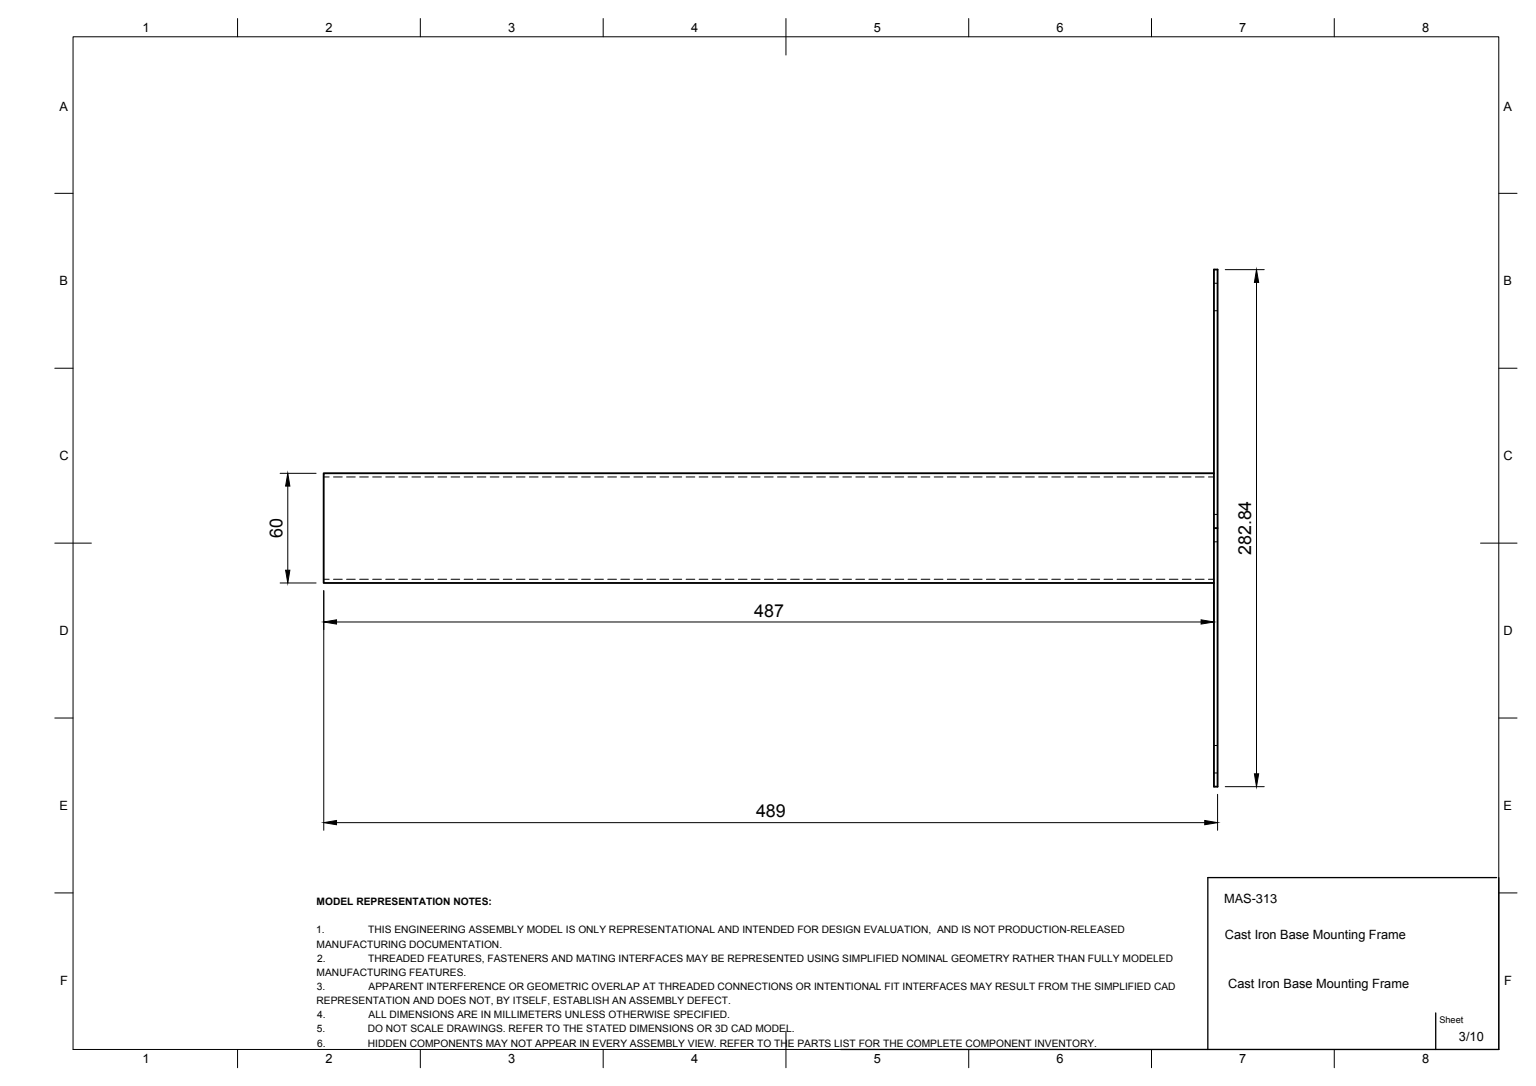
ISO-10303-21;
HEADER;
FILE_DESCRIPTION (('STEP AP214'),
    '1' );
FILE_NAME ('Cast Iron Base Mounting Frame.step',
    '2026-10-06T09:36:00',
    ( '' ),
    ( '' ),
    'SwSTEP 2.0',
    'SolidWorks 2025',
    '' );
FILE_SCHEMA (( 'AUTOMOTIVE_DESIGN' ));
ENDSEC;

DATA;
#2=ORIENTED_EDGE ( 'NONE', *, *, #7069, .T. ) ;
#13=CARTESIAN_POINT ( 'NONE',  ( -6.360897667028196044E-14, -494.9999999999998863, -141.4213562373094817 ) ) ;
#17=CYLINDRICAL_SURFACE ( 'NONE', #5203, 7.500000000000007105 ) ;
#40=DIRECTION ( 'NONE',  ( -6.195440985631454085E-17, 0.000000000000000000, 1.000000000000000000 ) ) ;
#61=CIRCLE ( 'NONE', #6581, 7.500000000000007105 ) ;
#73=LINE ( 'NONE', #6513, #3701 ) ;
#103=ORIENTED_EDGE ( 'NONE', *, *, #874, .T. ) ;
#112=DIRECTION ( 'NONE',  ( 1.000000000000000000, 0.000000000000000000, 0.000000000000000000 ) ) ;
#114=LINE ( 'NONE', #2966, #2548 ) ;
#160=AXIS2_PLACEMENT_3D ( 'NONE', #10271, #8167, #6559 ) ;
#171=CARTESIAN_POINT ( 'NONE',  ( -126.4213562373094959, -492.9999999999998863, 2.255140518769849223E-14 ) ) ;
#197=EDGE_LOOP ( 'NONE', ( #6499, #7897, #12076, #5197 ) ) ;
#203=ORIENTED_EDGE ( 'NONE', *, *, #874, .F. ) ;
#228=CARTESIAN_POINT ( 'NONE',  ( 0.000000000000000000, -494.9999999999998863, 0.000000000000000000 ) ) ;
#256=VECTOR ( 'NONE', #4482, 1000.000000000000000 ) ;
#258=LINE ( 'NONE', #2469, #6072 ) ;
#276=VECTOR ( 'NONE', #8146, 1000.000000000000000 ) ;
#358=ORIENTED_EDGE ( 'NONE', *, *, #9645, .T. ) ;
#376=CIRCLE ( 'NONE', #5908, 7.500000000000012434 ) ;
#381=DIRECTION ( 'NONE',  ( -0.000000000000000000, 1.000000000000000000, -0.000000000000000000 ) ) ;
#395=ORIENTED_EDGE ( 'NONE', *, *, #7971, .T. ) ;
#413=CARTESIAN_POINT ( 'NONE',  ( 1.387778780781445676E-14, -494.9999999999998863, 126.4213562373094959 ) ) ;
#429=CARTESIAN_POINT ( 'NONE',  ( 30.00000000000000000, -492.9999999999998863, -30.00000000000000000 ) ) ;
#436=FACE_OUTER_BOUND ( 'NONE', #2758, .T. ) ;
#507=CARTESIAN_POINT ( 'NONE',  ( -27.99999999999999645, -6.000000000000000000, 27.99999999999999645 ) ) ;
#510=PLANE ( 'NONE',  #8625 ) ;
#511=VECTOR ( 'NONE', #1443, 1000.000000000000000 ) ;
#532=VECTOR ( 'NONE', #8116, 1000.000000000000000 ) ;
#541=CARTESIAN_POINT ( 'NONE',  ( 4.808665244885994618E-14, -494.9999999999998863, 141.4213562373094817 ) ) ;
#558=SURFACE_STYLE_USAGE ( .BOTH. , #4395 ) ;
#565=FACE_OUTER_BOUND ( 'NONE', #10182, .T. ) ;
#577=CARTESIAN_POINT ( 'NONE',  ( 4.808665244885994618E-14, -492.9999999999998863, 141.4213562373094817 ) ) ;
#580=EDGE_CURVE ( 'NONE', #6384, #8630, #3180, .T. ) ;
#594=DIRECTION ( 'NONE',  ( -0.000000000000000000, 1.000000000000000000, -0.000000000000000000 ) ) ;
#623=FILL_AREA_STYLE ('',( #9083 ) ) ;
#628=ORIENTED_EDGE ( 'NONE', *, *, #11249, .F. ) ;
#657=LINE ( 'NONE', #9378, #2240 ) ;
#661=AXIS2_PLACEMENT_3D ( 'NONE', #11295, #2830, #6599 ) ;
#662=LINE ( 'NONE', #4437, #1336 ) ;
#665=DIRECTION ( 'NONE',  ( 0.7071067811865473507, 0.000000000000000000, -0.7071067811865477948 ) ) ;
#676=ORIENTED_EDGE ( 'NONE', *, *, #11233, .F. ) ;
#681=SURFACE_STYLE_FILL_AREA ( #9080 ) ;
#686=CARTESIAN_POINT ( 'NONE',  ( 1.387778780781445676E-14, -494.9999999999998863, 126.4213562373094959 ) ) ;
#706=CARTESIAN_POINT ( 'NONE',  ( 28.00000000000000000, -492.9999999999998863, -27.99999999999999645 ) ) ;
#730=EDGE_LOOP ( 'NONE', ( #10708, #628 ) ) ;
#752=( LENGTH_UNIT ( ) NAMED_UNIT ( * ) SI_UNIT ( .MILLI., .METRE. ) );
#755=DIRECTION ( 'NONE',  ( -0.000000000000000000, 1.000000000000000000, -0.000000000000000000 ) ) ;
#778=LINE ( 'NONE', #4551, #2867 ) ;
#781=DIRECTION ( 'NONE',  ( -0.000000000000000000, 1.000000000000000000, -0.000000000000000000 ) ) ;
#858=CARTESIAN_POINT ( 'NONE',  ( 141.4213562373095101, -494.9999999999998863, -1.508194112741312283E-14 ) ) ;
#874=EDGE_CURVE ( 'NONE', #6680, #11382, #2755, .T. ) ;
#882=VERTEX_POINT ( 'NONE', #9106 ) ;
#916=CARTESIAN_POINT ( 'NONE',  ( -27.99999999999999645, -492.9999999999998863, -27.99999999999999645 ) ) ;
#934=FACE_OUTER_BOUND ( 'NONE', #2126, .T. ) ;
#938=ORIENTED_EDGE ( 'NONE', *, *, #10249, .F. ) ;
#991=ORIENTED_EDGE ( 'NONE', *, *, #7995, .F. ) ;
#994=DIRECTION ( 'NONE',  ( 0.000000000000000000, -1.000000000000000000, 0.000000000000000000 ) ) ;
#1026=EDGE_CURVE ( 'NONE', #5299, #3186, #258, .T. ) ;
#1033=EDGE_LOOP ( 'NONE', ( #203, #3266, #1398, #1116 ) ) ;
#1034=AXIS2_PLACEMENT_3D ( 'NONE', #858, #4628, #3686 ) ;
#1048=ADVANCED_FACE ( 'NONE', ( #8799 ), #6941, .F. ) ;
#1055=CIRCLE ( 'NONE', #4008, 7.500000000000012434 ) ;
#1070=ORIENTED_EDGE ( 'NONE', *, *, #5111, .F. ) ;
#1081=ORIENTED_EDGE ( 'NONE', *, *, #7850, .T. ) ;
#1093=VECTOR ( 'NONE', #5863, 1000.000000000000000 ) ;
#1094=PRODUCT_CONTEXT ( 'NONE', #11592, 'mechanical' ) ;
#1095=VECTOR ( 'NONE', #2198, 1000.000000000000000 ) ;
#1116=ORIENTED_EDGE ( 'NONE', *, *, #10704, .F. ) ;
#1144=AXIS2_PLACEMENT_3D ( 'NONE', #1240, #7036, #2348 ) ;
#1159=STYLED_ITEM ( 'NONE', ( #3335 ), #8147 ) ;
#1160=CARTESIAN_POINT ( 'NONE',  ( -27.99999999999999645, -492.9999999999998863, -27.99999999999999645 ) ) ;
#1167=VERTEX_POINT ( 'NONE', #6427 ) ;
#1194=ORIENTED_EDGE ( 'NONE', *, *, #1790, .T. ) ;
#1207=CARTESIAN_POINT ( 'NONE',  ( 30.00000000000000000, -492.9999999999998863, 30.00000000000000000 ) ) ;
#1231=CIRCLE ( 'NONE', #8130, 7.500000000000007105 ) ;
#1236=FACE_BOUND ( 'NONE', #1923, .T. ) ;
#1238=CARTESIAN_POINT ( 'NONE',  ( -30.00000000000000000, -6.000000000000000000, 30.00000000000000000 ) ) ;
#1240=CARTESIAN_POINT ( 'NONE',  ( -126.4213562373094959, -494.9999999999998863, 2.255140518769849223E-14 ) ) ;
#1241=AXIS2_PLACEMENT_3D ( 'NONE', #6713, #7704, #3984 ) ;
#1245=LINE ( 'NONE', #6867, #3581 ) ;
#1255=CARTESIAN_POINT ( 'NONE',  ( 126.4213562373094959, -494.9999999999998863, 7.500000000000006217 ) ) ;
#1288=ORIENTED_EDGE ( 'NONE', *, *, #6220, .T. ) ;
#1334=DIRECTION ( 'NONE',  ( 0.000000000000000000, 0.000000000000000000, -1.000000000000000000 ) ) ;
#1336=VECTOR ( 'NONE', #3342, 1000.000000000000000 ) ;
#1342=VERTEX_POINT ( 'NONE', #7847 ) ;
#1349=( GEOMETRIC_REPRESENTATION_CONTEXT ( 3 ) GLOBAL_UNCERTAINTY_ASSIGNED_CONTEXT ( ( #11660 ) ) GLOBAL_UNIT_ASSIGNED_CONTEXT ( ( #752, #8169, #4338 ) ) REPRESENTATION_CONTEXT ( 'NONE', 'WORKASPACE' ) );
#1361=DIRECTION ( 'NONE',  ( -0.000000000000000000, 1.000000000000000000, -0.000000000000000000 ) ) ;
#1398=ORIENTED_EDGE ( 'NONE', *, *, #12116, .F. ) ;
#1443=DIRECTION ( 'NONE',  ( 1.000000000000000000, 0.000000000000000000, 0.000000000000000000 ) ) ;
#1450=VECTOR ( 'NONE', #6580, 1000.000000000000000 ) ;
#1463=VECTOR ( 'NONE', #10507, 1000.000000000000000 ) ;
#1470=LINE ( 'NONE', #4375, #276 ) ;
#1473=FACE_OUTER_BOUND ( 'NONE', #8723, .T. ) ;
#1477=LINE ( 'NONE', #11189, #6951 ) ;
#1480=EDGE_CURVE ( 'NONE', #6424, #6402, #662, .T. ) ;
#1481=DIRECTION ( 'NONE',  ( 0.000000000000000000, -1.000000000000000000, 0.000000000000000000 ) ) ;
#1495=EDGE_CURVE ( 'NONE', #2379, #1167, #5320, .T. ) ;
#1500=CARTESIAN_POINT ( 'NONE',  ( 1.387778780781445676E-14, -492.9999999999998863, 126.4213562373094959 ) ) ;
#1513=ORIENTED_EDGE ( 'NONE', *, *, #6743, .T. ) ;
#1514=CARTESIAN_POINT ( 'NONE',  ( 0.000000000000000000, -492.9999999999998863, 0.000000000000000000 ) ) ;
#1557=CARTESIAN_POINT ( 'NONE',  ( 4.808665244885994618E-14, -494.9999999999998863, 141.4213562373094817 ) ) ;
#1611=VERTEX_POINT ( 'NONE', #9641 ) ;
#1622=VERTEX_POINT ( 'NONE', #7855 ) ;
#1703=LINE ( 'NONE', #916, #11145 ) ;
#1735=VERTEX_POINT ( 'NONE', #12032 ) ;
#1737=ORIENTED_EDGE ( 'NONE', *, *, #7538, .T. ) ;
#1742=DIRECTION ( 'NONE',  ( -0.000000000000000000, 1.000000000000000000, -0.000000000000000000 ) ) ;
#1747=ORIENTED_EDGE ( 'NONE', *, *, #11277, .F. ) ;
#1790=EDGE_CURVE ( 'NONE', #7713, #882, #657, .T. ) ;
#1800=SURFACE_SIDE_STYLE ('',( #681 ) ) ;
#1817=ORIENTED_EDGE ( 'NONE', *, *, #9085, .F. ) ;
#1820=DIRECTION ( 'NONE',  ( 0.000000000000000000, 0.000000000000000000, -1.000000000000000000 ) ) ;
#1831=EDGE_LOOP ( 'NONE', ( #6682, #7432 ) ) ;
#1839=VECTOR ( 'NONE', #9227, 1000.000000000000000 ) ;
#1884=EDGE_CURVE ( 'NONE', #8131, #5617, #61, .T. ) ;
#1885=ORIENTED_EDGE ( 'NONE', *, *, #5319, .F. ) ;
#1917=DIRECTION ( 'NONE',  ( -0.000000000000000000, 0.000000000000000000, 1.000000000000000000 ) ) ;
#1921=CARTESIAN_POINT ( 'NONE',  ( 126.4213562373094959, -494.9999999999998863, -7.500000000000019540 ) ) ;
#1923=EDGE_LOOP ( 'NONE', ( #6325, #7312 ) ) ;
#1925=ORIENTED_EDGE ( 'NONE', *, *, #2302, .F. ) ;
#1928=DIRECTION ( 'NONE',  ( 0.000000000000000000, 0.000000000000000000, 1.000000000000000000 ) ) ;
#1941=DIRECTION ( 'NONE',  ( -0.7071067811865479058, 0.000000000000000000, -0.7071067811865472397 ) ) ;
#1963=DIRECTION ( 'NONE',  ( 0.000000000000000000, 0.000000000000000000, -1.000000000000000000 ) ) ;
#1970=CARTESIAN_POINT ( 'NONE',  ( 9.184850993605165694E-16, -494.9999999999998863, -133.9213562373095101 ) ) ;
#1982=DIRECTION ( 'NONE',  ( 0.000000000000000000, -0.000000000000000000, -1.000000000000000000 ) ) ;
#2015=VERTEX_POINT ( 'NONE', #9322 ) ;
#2037=FACE_BOUND ( 'NONE', #3887, .T. ) ;
#2060=DIRECTION ( 'NONE',  ( 0.7071067811865473507, 0.000000000000000000, -0.7071067811865477948 ) ) ;
#2061=VERTEX_POINT ( 'NONE', #1970 ) ;
#2067=VECTOR ( 'NONE', #10887, 1000.000000000000000 ) ;
#2083=ORIENTED_EDGE ( 'NONE', *, *, #9085, .T. ) ;
#2105=FACE_OUTER_BOUND ( 'NONE', #1033, .T. ) ;
#2120=CARTESIAN_POINT ( 'NONE',  ( -126.4213562373094959, -494.9999999999998863, 2.255140518769849223E-14 ) ) ;
#2122=VECTOR ( 'NONE', #2385, 999.9999999999998863 ) ;
#2126=EDGE_LOOP ( 'NONE', ( #1513, #11428, #1925, #8252 ) ) ;
#2138=ADVANCED_FACE ( 'NONE', ( #9503 ), #8580, .F. ) ;
#2141=VECTOR ( 'NONE', #2060, 999.9999999999998863 ) ;
#2153=AXIS2_PLACEMENT_3D ( 'NONE', #228, #994, #1982 ) ;
#2162=( GEOMETRIC_REPRESENTATION_CONTEXT ( 3 ) GLOBAL_UNCERTAINTY_ASSIGNED_CONTEXT ( ( #8812 ) ) GLOBAL_UNIT_ASSIGNED_CONTEXT ( ( #2722, #12126, #6304 ) ) REPRESENTATION_CONTEXT ( 'NONE', 'WORKASPACE' ) );
#2186=EDGE_LOOP ( 'NONE', ( #4571, #11548, #991, #8312 ) ) ;
#2198=DIRECTION ( 'NONE',  ( -0.000000000000000000, 1.000000000000000000, -0.000000000000000000 ) ) ;
#2240=VECTOR ( 'NONE', #11289, 1000.000000000000000 ) ;
#2247=CARTESIAN_POINT ( 'NONE',  ( -30.00000000000000000, -492.9999999999998863, -30.00000000000000000 ) ) ;
#2251=CARTESIAN_POINT ( 'NONE',  ( 126.4213562373094959, -492.9999999999998863, -6.938893903907228378E-15 ) ) ;
#2258=CIRCLE ( 'NONE', #5009, 7.500000000000012434 ) ;
#2267=EDGE_CURVE ( 'NONE', #3571, #7713, #9039, .T. ) ;
#2300=CARTESIAN_POINT ( 'NONE',  ( 28.00000000000000000, -492.9999999999998863, -27.99999999999999645 ) ) ;
#2302=EDGE_CURVE ( 'NONE', #6384, #5463, #8505, .T. ) ;
#2345=AXIS2_PLACEMENT_3D ( 'NONE', #1500, #10714, #5261 ) ;
#2348=DIRECTION ( 'NONE',  ( 0.000000000000000000, 0.000000000000000000, 1.000000000000000000 ) ) ;
#2379=VERTEX_POINT ( 'NONE', #13 ) ;
#2385=DIRECTION ( 'NONE',  ( 0.7071067811865479058, 0.000000000000000000, 0.7071067811865472397 ) ) ;
#2402=DIRECTION ( 'NONE',  ( -0.7071067811865473507, 0.000000000000000000, 0.7071067811865477948 ) ) ;
#2449=AXIS2_PLACEMENT_3D ( 'NONE', #4231, #4414, #1334 ) ;
#2469=CARTESIAN_POINT ( 'NONE',  ( 1.387778780781445676E-14, -494.9999999999998863, 133.9213562373095101 ) ) ;
#2548=VECTOR ( 'NONE', #6729, 1000.000000000000000 ) ;
#2554=CARTESIAN_POINT ( 'NONE',  ( 1.479627290717497352E-14, -494.9999999999998863, 118.9213562373094817 ) ) ;
#2562=CARTESIAN_POINT ( 'NONE',  ( 1.387778780781445676E-14, -494.9999999999998863, 126.4213562373094959 ) ) ;
#2586=DIRECTION ( 'NONE',  ( -0.000000000000000000, 1.000000000000000000, -0.000000000000000000 ) ) ;
#2591=CYLINDRICAL_SURFACE ( 'NONE', #8082, 7.500000000000007105 ) ;
#2627=CARTESIAN_POINT ( 'NONE',  ( -30.00000000000000000, -492.9999999999998863, 30.00000000000000000 ) ) ;
#2658=AXIS2_PLACEMENT_3D ( 'NONE', #4296, #3402, #8912 ) ;
#2662=FACE_BOUND ( 'NONE', #3396, .T. ) ;
#2674=CARTESIAN_POINT ( 'NONE',  ( -27.99999999999999645, -492.9999999999998863, -27.99999999999999645 ) ) ;
#2722=( LENGTH_UNIT ( ) NAMED_UNIT ( * ) SI_UNIT ( .MILLI., .METRE. ) );
#2745=VECTOR ( 'NONE', #11263, 1000.000000000000000 ) ;
#2755=LINE ( 'NONE', #5335, #9899 ) ;
#2758=EDGE_LOOP ( 'NONE', ( #6588, #8120, #3553, #10029 ) ) ;
#2796=EDGE_LOOP ( 'NONE', ( #4764, #9890, #7885, #7728 ) ) ;
#2830=DIRECTION ( 'NONE',  ( -0.000000000000000000, 1.000000000000000000, -0.000000000000000000 ) ) ;
#2860=FACE_OUTER_BOUND ( 'NONE', #11455, .T. ) ;
#2867=VECTOR ( 'NONE', #10231, 1000.000000000000000 ) ;
#2878=DIRECTION ( 'NONE',  ( -0.000000000000000000, 1.000000000000000000, -0.000000000000000000 ) ) ;
#2885=LINE ( 'NONE', #9490, #11176 ) ;
#2886=DIRECTION ( 'NONE',  ( 0.000000000000000000, -1.000000000000000000, 0.000000000000000000 ) ) ;
#2892=( GEOMETRIC_REPRESENTATION_CONTEXT ( 3 ) GLOBAL_UNCERTAINTY_ASSIGNED_CONTEXT ( ( #9795 ) ) GLOBAL_UNIT_ASSIGNED_CONTEXT ( ( #4176, #6096, #3300 ) ) REPRESENTATION_CONTEXT ( 'NONE', 'WORKASPACE' ) );
#2910=PLANE ( 'NONE',  #10244 ) ;
#2912=PLANE ( 'NONE',  #3232 ) ;
#2919=EDGE_LOOP ( 'NONE', ( #12184, #7238, #7706, #2 ) ) ;
#2966=CARTESIAN_POINT ( 'NONE',  ( 141.4213562373095101, -494.9999999999998863, -1.508194112741312283E-14 ) ) ;
#2973=CARTESIAN_POINT ( 'NONE',  ( 1.387778780781445676E-14, -494.9999999999998863, 126.4213562373094959 ) ) ;
#3032=ORIENTED_EDGE ( 'NONE', *, *, #6284, .F. ) ;
#3043=ORIENTED_EDGE ( 'NONE', *, *, #9421, .F. ) ;
#3060=VECTOR ( 'NONE', #8488, 1000.000000000000000 ) ;
#3086=VECTOR ( 'NONE', #6084, 1000.000000000000000 ) ;
#3131=EDGE_LOOP ( 'NONE', ( #3257, #6840, #1194, #11050 ) ) ;
#3139=COLOUR_RGB ( '', 0.66274510, 0.83137255, 0.94901961) ;
#3143=PRODUCT_DEFINITION ( 'UNKNOWN', '', #3878, #11351 ) ;
#3180=LINE ( 'NONE', #5271, #7532 ) ;
#3186=VERTEX_POINT ( 'NONE', #5560 ) ;
#3200=DIRECTION ( 'NONE',  ( 0.000000000000000000, 0.000000000000000000, 1.000000000000000000 ) ) ;
#3232=AXIS2_PLACEMENT_3D ( 'NONE', #11313, #10567, #3892 ) ;
#3257=ORIENTED_EDGE ( 'NONE', *, *, #4672, .F. ) ;
#3266=ORIENTED_EDGE ( 'NONE', *, *, #10375, .F. ) ;
#3273=CARTESIAN_POINT ( 'NONE',  ( 0.000000000000000000, -492.9999999999998863, -126.4213562373094959 ) ) ;
#3279=ORIENTED_EDGE ( 'NONE', *, *, #6743, .F. ) ;
#3289=ADVANCED_FACE ( 'NONE', ( #934 ), #4706, .F. ) ;
#3294=CARTESIAN_POINT ( 'NONE',  ( -27.99999999999999645, -492.9999999999998863, -27.99999999999999645 ) ) ;
#3298=EDGE_LOOP ( 'NONE', ( #1885, #8268, #8263, #10866 ) ) ;
#3300=( NAMED_UNIT ( * ) SI_UNIT ( $, .STERADIAN. ) SOLID_ANGLE_UNIT ( ) );
#3303=DIRECTION ( 'NONE',  ( 0.000000000000000000, -1.000000000000000000, 0.000000000000000000 ) ) ;
#3317=CARTESIAN_POINT ( 'NONE',  ( 30.00000000000000000, -6.000000000000000000, 30.00000000000000000 ) ) ;
#3324=STYLED_ITEM ( 'NONE', ( #9337 ), #3758 ) ;
#3335=PRESENTATION_STYLE_ASSIGNMENT (( #558 ) ) ;
#3342=DIRECTION ( 'NONE',  ( -0.000000000000000000, 1.000000000000000000, -0.000000000000000000 ) ) ;
#3343=CARTESIAN_POINT ( 'NONE',  ( 28.00000000000000000, -492.9999999999998863, -27.99999999999999645 ) ) ;
#3367=AXIS2_PLACEMENT_3D ( 'NONE', #11658, #6029, #9911 ) ;
#3373=DIRECTION ( 'NONE',  ( 0.7071067811865477948, 0.000000000000000000, 0.7071067811865473507 ) ) ;
#3376=AXIS2_PLACEMENT_3D ( 'NONE', #4147, #5182, #6056 ) ;
#3389=ORIENTED_EDGE ( 'NONE', *, *, #5441, .F. ) ;
#3393=ADVANCED_FACE ( 'NONE', ( #2037, #4871, #9456, #3826, #4934 ), #9578, .T. ) ;
#3394=DIRECTION ( 'NONE',  ( 0.000000000000000000, 0.000000000000000000, 1.000000000000000000 ) ) ;
#3396=EDGE_LOOP ( 'NONE', ( #10120, #11963, #11935, #1737 ) ) ;
#3402=DIRECTION ( 'NONE',  ( 0.000000000000000000, -1.000000000000000000, 0.000000000000000000 ) ) ;
#3414=CARTESIAN_POINT ( 'NONE',  ( 1.387778780781445676E-14, -492.9999999999998863, 126.4213562373094959 ) ) ;
#3437=ADVANCED_FACE ( 'NONE', ( #2105, #11370, #6857, #8771, #1236 ), #2910, .F. ) ;
#3439=VECTOR ( 'NONE', #4347, 1000.000000000000000 ) ;
#3445=ORIENTED_EDGE ( 'NONE', *, *, #2302, .T. ) ;
#3458=ORIENTED_EDGE ( 'NONE', *, *, #1480, .T. ) ;
#3466=CIRCLE ( 'NONE', #6450, 7.500000000000012434 ) ;
#3470=CARTESIAN_POINT ( 'NONE',  ( 30.00000000000000000, -6.000000000000000000, -30.00000000000000000 ) ) ;
#3553=ORIENTED_EDGE ( 'NONE', *, *, #2267, .T. ) ;
#3571=VERTEX_POINT ( 'NONE', #8935 ) ;
#3581=VECTOR ( 'NONE', #11319, 1000.000000000000000 ) ;
#3588=LINE ( 'NONE', #2674, #1839 ) ;
#3601=SHAPE_REPRESENTATION ( 'Cast Iron Base Mounting Frame', ( #11957 ), #2892 ) ;
#3619=CARTESIAN_POINT ( 'NONE',  ( 4.808665244885994618E-14, -494.9999999999998863, 141.4213562373094817 ) ) ;
#3686=DIRECTION ( 'NONE',  ( -0.7071067811865473507, 0.000000000000000000, 0.7071067811865477948 ) ) ;
#3700=ORIENTED_EDGE ( 'NONE', *, *, #10907, .F. ) ;
#3701=VECTOR ( 'NONE', #3851, 999.9999999999998863 ) ;
#3754=ADVANCED_FACE ( 'NONE', ( #4334 ), #2591, .F. ) ;
#3758=MANIFOLD_SOLID_BREP ( 'Boss-Extrude7', #9857 ) ;
#3777=ORIENTED_EDGE ( 'NONE', *, *, #7850, .F. ) ;
#3815=ORIENTED_EDGE ( 'NONE', *, *, #7386, .T. ) ;
#3826=FACE_BOUND ( 'NONE', #7708, .T. ) ;
#3830=ADVANCED_BREP_SHAPE_REPRESENTATION ( '', ( #3758, #8147, #11957 ), #2892 ) ;
#3838=EDGE_LOOP ( 'NONE', ( #9982, #11366, #11265, #4376 ) ) ;
#3851=DIRECTION ( 'NONE',  ( 0.7071067811865479058, 0.000000000000000000, 0.7071067811865472397 ) ) ;
#3869=LINE ( 'NONE', #7761, #8276 ) ;
#3878=PRODUCT_DEFINITION_FORMATION_WITH_SPECIFIED_SOURCE ( 'ANY', '', #8619, .NOT_KNOWN. ) ;
#3879=ORIENTED_EDGE ( 'NONE', *, *, #1026, .F. ) ;
#3887=EDGE_LOOP ( 'NONE', ( #9683, #1817 ) ) ;
#3892=DIRECTION ( 'NONE',  ( -1.000000000000000000, 0.000000000000000000, -6.195440985631454085E-17 ) ) ;
#3893=ORIENTED_EDGE ( 'NONE', *, *, #5543, .T. ) ;
#3917=ORIENTED_EDGE ( 'NONE', *, *, #9408, .T. ) ;
#3918=EDGE_LOOP ( 'NONE', ( #5642, #3917 ) ) ;
#3922=ORIENTED_EDGE ( 'NONE', *, *, #6903, .F. ) ;
#3959=EDGE_CURVE ( 'NONE', #10867, #6680, #114, .T. ) ;
#3978=EDGE_CURVE ( 'NONE', #6402, #8803, #376, .T. ) ;
#3984=DIRECTION ( 'NONE',  ( 0.000000000000000000, 0.000000000000000000, -1.000000000000000000 ) ) ;
#4008=AXIS2_PLACEMENT_3D ( 'NONE', #2251, #10833, #6020 ) ;
#4080=VECTOR ( 'NONE', #381, 1000.000000000000000 ) ;
#4123=EDGE_CURVE ( 'NONE', #3186, #1611, #8088, .T. ) ;
#4124=ORIENTED_EDGE ( 'NONE', *, *, #6843, .F. ) ;
#4147=CARTESIAN_POINT ( 'NONE',  ( -126.4213562373094959, -494.9999999999998863, 2.255140518769849223E-14 ) ) ;
#4176=( LENGTH_UNIT ( ) NAMED_UNIT ( * ) SI_UNIT ( .MILLI., .METRE. ) );
#4221=CARTESIAN_POINT ( 'NONE',  ( 141.4213562373095101, -494.9999999999998863, -1.508194112741312283E-14 ) ) ;
#4231=CARTESIAN_POINT ( 'NONE',  ( 0.000000000000000000, -494.9999999999998863, -126.4213562373094959 ) ) ;
#4233=LINE ( 'NONE', #3294, #511 ) ;
#4239=AXIS2_PLACEMENT_3D ( 'NONE', #11561, #3303, #5162 ) ;
#4296=CARTESIAN_POINT ( 'NONE',  ( -126.4213562373094959, -492.9999999999998863, 2.255140518769849223E-14 ) ) ;
#4305=FACE_BOUND ( 'NONE', #197, .T. ) ;
#4321=AXIS2_PLACEMENT_3D ( 'NONE', #686, #6436, #8367 ) ;
#4334=FACE_OUTER_BOUND ( 'NONE', #8748, .T. ) ;
#4338=( NAMED_UNIT ( * ) SI_UNIT ( $, .STERADIAN. ) SOLID_ANGLE_UNIT ( ) );
#4345=CYLINDRICAL_SURFACE ( 'NONE', #8030, 7.500000000000012434 ) ;
#4347=DIRECTION ( 'NONE',  ( -0.000000000000000000, -0.000000000000000000, -1.000000000000000000 ) ) ;
#4359=CARTESIAN_POINT ( 'NONE',  ( 28.00000000000000000, -6.000000000000000000, -27.99999999999999645 ) ) ;
#4365=ORIENTED_EDGE ( 'NONE', *, *, #10907, .T. ) ;
#4375=CARTESIAN_POINT ( 'NONE',  ( -27.99999999999999645, -6.000000000000000000, -27.99999999999999645 ) ) ;
#4376=ORIENTED_EDGE ( 'NONE', *, *, #10779, .T. ) ;
#4395=SURFACE_SIDE_STYLE ('',( #10877 ) ) ;
#4401=EDGE_CURVE ( 'NONE', #4868, #10168, #11965, .T. ) ;
#4414=DIRECTION ( 'NONE',  ( 0.000000000000000000, -1.000000000000000000, 0.000000000000000000 ) ) ;
#4437=CARTESIAN_POINT ( 'NONE',  ( -126.4213562373094959, -494.9999999999998863, -7.499999999999990230 ) ) ;
#4442=LINE ( 'NONE', #11916, #5050 ) ;
#4459=ORIENTED_EDGE ( 'NONE', *, *, #1495, .F. ) ;
#4482=DIRECTION ( 'NONE',  ( -6.195440985631455317E-17, 0.000000000000000000, 1.000000000000000000 ) ) ;
#4503=ORIENTED_EDGE ( 'NONE', *, *, #8108, .F. ) ;
#4505=FACE_OUTER_BOUND ( 'NONE', #3838, .T. ) ;
#4508=FACE_OUTER_BOUND ( 'NONE', #5762, .T. ) ;
#4512=EDGE_CURVE ( 'NONE', #882, #10332, #3869, .T. ) ;
#4528=ORIENTED_EDGE ( 'NONE', *, *, #6284, .T. ) ;
#4539=LINE ( 'NONE', #1557, #532 ) ;
#4551=CARTESIAN_POINT ( 'NONE',  ( 30.00000000000000000, -492.9999999999998863, -30.00000000000000000 ) ) ;
#4571=ORIENTED_EDGE ( 'NONE', *, *, #10375, .T. ) ;
#4576=CARTESIAN_POINT ( 'NONE',  ( -141.4213562373095101, -494.9999999999998863, 3.644282033693712520E-14 ) ) ;
#4581=VERTEX_POINT ( 'NONE', #1160 ) ;
#4628=DIRECTION ( 'NONE',  ( -0.7071067811865477948, 0.000000000000000000, -0.7071067811865473507 ) ) ;
#4642=AXIS2_PLACEMENT_3D ( 'NONE', #3414, #6154, #8075 ) ;
#4645=EDGE_CURVE ( 'NONE', #1342, #2015, #6742, .T. ) ;
#4653=VECTOR ( 'NONE', #5823, 1000.000000000000000 ) ;
#4662=ORIENTED_EDGE ( 'NONE', *, *, #580, .F. ) ;
#4672=EDGE_CURVE ( 'NONE', #9067, #10332, #7843, .T. ) ;
#4706=PLANE ( 'NONE',  #12225 ) ;
#4725=LINE ( 'NONE', #5817, #5195 ) ;
#4728=LINE ( 'NONE', #11220, #11006 ) ;
#4739=ORIENTED_EDGE ( 'NONE', *, *, #4401, .F. ) ;
#4764=ORIENTED_EDGE ( 'NONE', *, *, #5752, .T. ) ;
#4785=CIRCLE ( 'NONE', #3376, 7.500000000000012434 ) ;
#4866=ADVANCED_FACE ( 'NONE', ( #12170 ), #11241, .F. ) ;
#4868=VERTEX_POINT ( 'NONE', #8406 ) ;
#4871=FACE_BOUND ( 'NONE', #730, .T. ) ;
#4889=MECHANICAL_DESIGN_GEOMETRIC_PRESENTATION_REPRESENTATION('',(#1159),#1349);
#4934=FACE_BOUND ( 'NONE', #8354, .T. ) ;
#4952=ADVANCED_FACE ( 'NONE', ( #5180 ), #7918, .F. ) ;
#4970=EDGE_LOOP ( 'NONE', ( #7452, #395, #1081, #10447 ) ) ;
#4994=DIRECTION ( 'NONE',  ( -1.000000000000000000, -0.000000000000000000, -0.000000000000000000 ) ) ;
#5009=AXIS2_PLACEMENT_3D ( 'NONE', #2120, #5879, #9658 ) ;
#5045=CARTESIAN_POINT ( 'NONE',  ( -27.99999999999999645, -6.000000000000000000, 27.99999999999999645 ) ) ;
#5050=VECTOR ( 'NONE', #10988, 1000.000000000000000 ) ;
#5059=LINE ( 'NONE', #7104, #9328 ) ;
#5062=ORIENTED_EDGE ( 'NONE', *, *, #1884, .T. ) ;
#5072=LINE ( 'NONE', #5881, #6076 ) ;
#5077=LINE ( 'NONE', #429, #4080 ) ;
#5111=EDGE_CURVE ( 'NONE', #10867, #11480, #1477, .T. ) ;
#5139=ORIENTED_EDGE ( 'NONE', *, *, #11277, .T. ) ;
#5143=ORIENTED_EDGE ( 'NONE', *, *, #9340, .F. ) ;
#5156=ADVANCED_FACE ( 'NONE', ( #4508 ), #6237, .F. ) ;
#5162=DIRECTION ( 'NONE',  ( 0.000000000000000000, 0.000000000000000000, -1.000000000000000000 ) ) ;
#5180=FACE_OUTER_BOUND ( 'NONE', #6618, .T. ) ;
#5182=DIRECTION ( 'NONE',  ( 0.000000000000000000, -1.000000000000000000, 0.000000000000000000 ) ) ;
#5193=VERTEX_POINT ( 'NONE', #4576 ) ;
#5195=VECTOR ( 'NONE', #7622, 1000.000000000000000 ) ;
#5197=ORIENTED_EDGE ( 'NONE', *, *, #9793, .F. ) ;
#5203=AXIS2_PLACEMENT_3D ( 'NONE', #5766, #2878, #5891 ) ;
#5261=DIRECTION ( 'NONE',  ( 0.000000000000000000, 0.000000000000000000, -1.000000000000000000 ) ) ;
#5264=FACE_OUTER_BOUND ( 'NONE', #8950, .T. ) ;
#5271=CARTESIAN_POINT ( 'NONE',  ( -30.00000000000000000, -492.9999999999998863, -30.00000000000000000 ) ) ;
#5276=DIRECTION ( 'NONE',  ( 0.000000000000000000, 1.000000000000000000, 0.000000000000000000 ) ) ;
#5289=PLANE ( 'NONE',  #9372 ) ;
#5299=VERTEX_POINT ( 'NONE', #9587 ) ;
#5307=ADVANCED_FACE ( 'NONE', ( #2860 ), #8543, .F. ) ;
#5319=EDGE_CURVE ( 'NONE', #6347, #10683, #1245, .T. ) ;
#5320=LINE ( 'NONE', #9965, #5588 ) ;
#5328=PLANE ( 'NONE',  #5675 ) ;
#5335=CARTESIAN_POINT ( 'NONE',  ( 141.4213562373095101, -492.9999999999998863, -1.508194112741312283E-14 ) ) ;
#5441=EDGE_CURVE ( 'NONE', #11262, #9215, #5059, .T. ) ;
#5463=VERTEX_POINT ( 'NONE', #8040 ) ;
#5474=AXIS2_PLACEMENT_3D ( 'NONE', #2247, #11990, #9782 ) ;
#5488=ADVANCED_FACE ( 'NONE', ( #7041 ), #8889, .F. ) ;
#5509=ORIENTED_EDGE ( 'NONE', *, *, #8908, .F. ) ;
#5525=CARTESIAN_POINT ( 'NONE',  ( -30.00000000000000000, -492.9999999999998863, -30.00000000000000000 ) ) ;
#5543=EDGE_CURVE ( 'NONE', #6424, #1735, #4785, .T. ) ;
#5555=EDGE_CURVE ( 'NONE', #5299, #7650, #1231, .T. ) ;
#5560=CARTESIAN_POINT ( 'NONE',  ( 1.387778780781445676E-14, -492.9999999999998863, 133.9213562373095101 ) ) ;
#5562=SURFACE_STYLE_USAGE ( .BOTH. , #1800 ) ;
#5588=VECTOR ( 'NONE', #7185, 1000.000000000000000 ) ;
#5608=EDGE_LOOP ( 'NONE', ( #103, #11015, #1070, #9434 ) ) ;
#5617=VERTEX_POINT ( 'NONE', #12101 ) ;
#5642=ORIENTED_EDGE ( 'NONE', *, *, #5852, .T. ) ;
#5675=AXIS2_PLACEMENT_3D ( 'NONE', #7255, #1820, #7685 ) ;
#5718=DIRECTION ( 'NONE',  ( 0.000000000000000000, 0.000000000000000000, -1.000000000000000000 ) ) ;
#5739=DIRECTION ( 'NONE',  ( 0.000000000000000000, -0.000000000000000000, -1.000000000000000000 ) ) ;
#5743=CARTESIAN_POINT ( 'NONE',  ( 141.4213562373095101, -492.9999999999998863, -1.508194112741312283E-14 ) ) ;
#5752=EDGE_CURVE ( 'NONE', #11517, #2061, #8361, .T. ) ;
#5761=AXIS2_PLACEMENT_3D ( 'NONE', #11982, #3373, #10929 ) ;
#5762=EDGE_LOOP ( 'NONE', ( #10342, #4459, #3777, #1288 ) ) ;
#5766=CARTESIAN_POINT ( 'NONE',  ( 0.000000000000000000, -494.9999999999998863, -126.4213562373094959 ) ) ;
#5770=CARTESIAN_POINT ( 'NONE',  ( -126.4213562373094959, -492.9999999999998863, 7.500000000000035527 ) ) ;
#5787=CARTESIAN_POINT ( 'NONE',  ( -30.00000000000000000, -6.000000000000000000, -30.00000000000000000 ) ) ;
#5817=CARTESIAN_POINT ( 'NONE',  ( -141.4213562373095101, -494.9999999999998863, 3.644282033693712520E-14 ) ) ;
#5822=VECTOR ( 'NONE', #4994, 1000.000000000000000 ) ;
#5823=DIRECTION ( 'NONE',  ( -0.000000000000000000, 1.000000000000000000, -0.000000000000000000 ) ) ;
#5825=ORIENTED_EDGE ( 'NONE', *, *, #5543, .F. ) ;
#5831=LINE ( 'NONE', #10654, #11552 ) ;
#5840=DIRECTION ( 'NONE',  ( -0.000000000000000000, 1.000000000000000000, -0.000000000000000000 ) ) ;
#5852=EDGE_CURVE ( 'NONE', #7207, #1622, #1055, .T. ) ;
#5863=DIRECTION ( 'NONE',  ( 1.000000000000000000, 0.000000000000000000, 0.000000000000000000 ) ) ;
#5879=DIRECTION ( 'NONE',  ( 0.000000000000000000, -1.000000000000000000, 0.000000000000000000 ) ) ;
#5881=CARTESIAN_POINT ( 'NONE',  ( 9.184850993605161750E-16, -494.9999999999998863, -133.9213562373095101 ) ) ;
#5891=DIRECTION ( 'NONE',  ( 0.000000000000000000, 0.000000000000000000, 1.000000000000000000 ) ) ;
#5895=DIRECTION ( 'NONE',  ( -6.195440985631455317E-17, 0.000000000000000000, 1.000000000000000000 ) ) ;
#5908=AXIS2_PLACEMENT_3D ( 'NONE', #171, #7720, #11495 ) ;
#5974=ORIENTED_EDGE ( 'NONE', *, *, #8854, .F. ) ;
#6004=AXIS2_PLACEMENT_3D ( 'NONE', #9338, #12192, #9143 ) ;
#6009=PLANE ( 'NONE',  #10594 ) ;
#6017=LINE ( 'NONE', #3343, #2067 ) ;
#6020=DIRECTION ( 'NONE',  ( 0.000000000000000000, 0.000000000000000000, -1.000000000000000000 ) ) ;
#6029=DIRECTION ( 'NONE',  ( 0.000000000000000000, -1.000000000000000000, 0.000000000000000000 ) ) ;
#6031=EDGE_CURVE ( 'NONE', #882, #4581, #3588, .T. ) ;
#6056=DIRECTION ( 'NONE',  ( 0.000000000000000000, 0.000000000000000000, -1.000000000000000000 ) ) ;
#6072=VECTOR ( 'NONE', #2586, 1000.000000000000000 ) ;
#6076=VECTOR ( 'NONE', #8848, 1000.000000000000000 ) ;
#6084=DIRECTION ( 'NONE',  ( -0.000000000000000000, 1.000000000000000000, -0.000000000000000000 ) ) ;
#6096=( NAMED_UNIT ( * ) PLANE_ANGLE_UNIT ( ) SI_UNIT ( $, .RADIAN. ) );
#6139=ORIENTED_EDGE ( 'NONE', *, *, #5441, .T. ) ;
#6154=DIRECTION ( 'NONE',  ( 0.000000000000000000, -1.000000000000000000, 0.000000000000000000 ) ) ;
#6194=ORIENTED_EDGE ( 'NONE', *, *, #4401, .T. ) ;
#6204=ORIENTED_EDGE ( 'NONE', *, *, #9340, .T. ) ;
#6220=EDGE_CURVE ( 'NONE', #5193, #7316, #4725, .T. ) ;
#6237=PLANE ( 'NONE',  #5761 ) ;
#6248=DIRECTION ( 'NONE',  ( 0.000000000000000000, 0.000000000000000000, 1.000000000000000000 ) ) ;
#6271=CARTESIAN_POINT ( 'NONE',  ( 4.808665244885994618E-14, -492.9999999999998863, 141.4213562373094817 ) ) ;
#6284=EDGE_CURVE ( 'NONE', #1735, #6424, #2258, .T. ) ;
#6304=( NAMED_UNIT ( * ) SI_UNIT ( $, .STERADIAN. ) SOLID_ANGLE_UNIT ( ) );
#6325=ORIENTED_EDGE ( 'NONE', *, *, #11233, .T. ) ;
#6347=VERTEX_POINT ( 'NONE', #11760 ) ;
#6364=FACE_OUTER_BOUND ( 'NONE', #3131, .T. ) ;
#6368=CARTESIAN_POINT ( 'NONE',  ( 0.000000000000000000, -492.9999999999998863, -118.9213562373094817 ) ) ;
#6384=VERTEX_POINT ( 'NONE', #10943 ) ;
#6402=VERTEX_POINT ( 'NONE', #10700 ) ;
#6424=VERTEX_POINT ( 'NONE', #10819 ) ;
#6427=CARTESIAN_POINT ( 'NONE',  ( -6.360897667028196044E-14, -492.9999999999998863, -141.4213562373094817 ) ) ;
#6436=DIRECTION ( 'NONE',  ( 0.000000000000000000, -1.000000000000000000, 0.000000000000000000 ) ) ;
#6441=ORIENTED_EDGE ( 'NONE', *, *, #4123, .F. ) ;
#6450=AXIS2_PLACEMENT_3D ( 'NONE', #11345, #2886, #5718 ) ;
#6499=ORIENTED_EDGE ( 'NONE', *, *, #6031, .F. ) ;
#6513=CARTESIAN_POINT ( 'NONE',  ( -6.360897667028196044E-14, -494.9999999999998863, -141.4213562373094817 ) ) ;
#6559=DIRECTION ( 'NONE',  ( 0.000000000000000000, -0.000000000000000000, 1.000000000000000000 ) ) ;
#6572=ORIENTED_EDGE ( 'NONE', *, *, #1480, .F. ) ;
#6580=DIRECTION ( 'NONE',  ( 1.000000000000000000, 0.000000000000000000, 0.000000000000000000 ) ) ;
#6581=AXIS2_PLACEMENT_3D ( 'NONE', #6653, #10423, #1963 ) ;
#6588=ORIENTED_EDGE ( 'NONE', *, *, #7538, .F. ) ;
#6596=ADVANCED_FACE ( 'NONE', ( #10073 ), #8302, .T. ) ;
#6599=DIRECTION ( 'NONE',  ( 0.000000000000000000, 0.000000000000000000, 1.000000000000000000 ) ) ;
#6607=CIRCLE ( 'NONE', #4642, 7.500000000000007105 ) ;
#6616=LINE ( 'NONE', #7785, #1093 ) ;
#6618=EDGE_LOOP ( 'NONE', ( #4528, #3458, #676, #938 ) ) ;
#6623=DIRECTION ( 'NONE',  ( -0.000000000000000000, 1.000000000000000000, -0.000000000000000000 ) ) ;
#6653=CARTESIAN_POINT ( 'NONE',  ( 0.000000000000000000, -492.9999999999998863, -126.4213562373094959 ) ) ;
#6667=ADVANCED_FACE ( 'NONE', ( #6364 ), #2912, .T. ) ;
#6680=VERTEX_POINT ( 'NONE', #5743 ) ;
#6682=ORIENTED_EDGE ( 'NONE', *, *, #4123, .T. ) ;
#6713=CARTESIAN_POINT ( 'NONE',  ( 0.000000000000000000, -494.9999999999998863, -126.4213562373094959 ) ) ;
#6729=DIRECTION ( 'NONE',  ( -0.000000000000000000, 1.000000000000000000, -0.000000000000000000 ) ) ;
#6742=CIRCLE ( 'NONE', #3367, 7.500000000000012434 ) ;
#6743=EDGE_CURVE ( 'NONE', #8630, #11262, #6616, .T. ) ;
#6840=ORIENTED_EDGE ( 'NONE', *, *, #11739, .F. ) ;
#6843=EDGE_CURVE ( 'NONE', #2015, #1622, #11372, .T. ) ;
#6857=FACE_BOUND ( 'NONE', #3918, .T. ) ;
#6867=CARTESIAN_POINT ( 'NONE',  ( -27.99999999999999645, -6.000000000000000000, -27.99999999999999645 ) ) ;
#6891=EDGE_LOOP ( 'NONE', ( #3815, #4662, #5509, #6194 ) ) ;
#6903=EDGE_CURVE ( 'NONE', #1611, #3186, #6607, .T. ) ;
#6937=EDGE_CURVE ( 'NONE', #2015, #1342, #10942, .T. ) ;
#6941=PLANE ( 'NONE',  #5474 ) ;
#6942=FACE_OUTER_BOUND ( 'NONE', #3298, .T. ) ;
#6951=VECTOR ( 'NONE', #11918, 999.9999999999998863 ) ;
#6987=ADVANCED_FACE ( 'NONE', ( #9985, #4305 ), #11896, .F. ) ;
#7036=DIRECTION ( 'NONE',  ( -0.000000000000000000, 1.000000000000000000, -0.000000000000000000 ) ) ;
#7041=FACE_OUTER_BOUND ( 'NONE', #2186, .T. ) ;
#7069=EDGE_CURVE ( 'NONE', #4581, #6347, #1703, .T. ) ;
#7104=CARTESIAN_POINT ( 'NONE',  ( 30.00000000000000000, -6.000000000000000000, -30.00000000000000000 ) ) ;
#7130=LINE ( 'NONE', #8064, #9373 ) ;
#7143=ADVANCED_FACE ( 'NONE', ( #4505 ), #5289, .F. ) ;
#7166=DIRECTION ( 'NONE',  ( 0.000000000000000000, 0.000000000000000000, 1.000000000000000000 ) ) ;
#7185=DIRECTION ( 'NONE',  ( -0.000000000000000000, 1.000000000000000000, -0.000000000000000000 ) ) ;
#7191=EDGE_CURVE ( 'NONE', #10332, #6347, #1470, .T. ) ;
#7207=VERTEX_POINT ( 'NONE', #11468 ) ;
#7238=ORIENTED_EDGE ( 'NONE', *, *, #4512, .F. ) ;
#7242=CARTESIAN_POINT ( 'NONE',  ( -30.00000000000000000, -6.000000000000000000, 30.00000000000000000 ) ) ;
#7255=CARTESIAN_POINT ( 'NONE',  ( -30.00000000000000000, -492.9999999999998863, 30.00000000000000000 ) ) ;
#7274=CIRCLE ( 'NONE', #4321, 7.500000000000007105 ) ;
#7306=PLANE ( 'NONE',  #160 ) ;
#7312=ORIENTED_EDGE ( 'NONE', *, *, #3978, .T. ) ;
#7314=LINE ( 'NONE', #12073, #3439 ) ;
#7316=VERTEX_POINT ( 'NONE', #10206 ) ;
#7323=LINE ( 'NONE', #1255, #4653 ) ;
#7339=VECTOR ( 'NONE', #11791, 1000.000000000000000 ) ;
#7349=AXIS2_PLACEMENT_3D ( 'NONE', #2973, #6623, #1928 ) ;
#7350=ADVANCED_FACE ( 'NONE', ( #9699 ), #12025, .F. ) ;
#7360=FILL_AREA_STYLE_COLOUR ( '', #3139 ) ;
#7386=EDGE_CURVE ( 'NONE', #10168, #8630, #7314, .T. ) ;
#7432=ORIENTED_EDGE ( 'NONE', *, *, #6903, .T. ) ;
#7452=ORIENTED_EDGE ( 'NONE', *, *, #5111, .T. ) ;
#7468=ORIENTED_EDGE ( 'NONE', *, *, #6937, .F. ) ;
#7532=VECTOR ( 'NONE', #7830, 1000.000000000000000 ) ;
#7533=CARTESIAN_POINT ( 'NONE',  ( -126.4213562373094959, -494.9999999999998863, 7.500000000000035527 ) ) ;
#7538=EDGE_CURVE ( 'NONE', #10683, #9067, #5831, .T. ) ;
#7622=DIRECTION ( 'NONE',  ( -0.000000000000000000, 1.000000000000000000, -0.000000000000000000 ) ) ;
#7650=VERTEX_POINT ( 'NONE', #2554 ) ;
#7685=DIRECTION ( 'NONE',  ( -1.000000000000000000, 0.000000000000000000, -0.000000000000000000 ) ) ;
#7704=DIRECTION ( 'NONE',  ( 0.000000000000000000, -1.000000000000000000, 0.000000000000000000 ) ) ;
#7706=ORIENTED_EDGE ( 'NONE', *, *, #6031, .T. ) ;
#7708=EDGE_LOOP ( 'NONE', ( #9690, #7468 ) ) ;
#7713=VERTEX_POINT ( 'NONE', #9298 ) ;
#7720=DIRECTION ( 'NONE',  ( 0.000000000000000000, -1.000000000000000000, 0.000000000000000000 ) ) ;
#7728=ORIENTED_EDGE ( 'NONE', *, *, #11081, .F. ) ;
#7752=EDGE_LOOP ( 'NONE', ( #3043, #2083, #9599, #3922 ) ) ;
#7761=CARTESIAN_POINT ( 'NONE',  ( -27.99999999999999645, -492.9999999999998863, 27.99999999999999645 ) ) ;
#7785=CARTESIAN_POINT ( 'NONE',  ( -30.00000000000000000, -6.000000000000000000, -30.00000000000000000 ) ) ;
#7786=ORIENTED_EDGE ( 'NONE', *, *, #5852, .F. ) ;
#7790=CIRCLE ( 'NONE', #2449, 7.500000000000007105 ) ;
#7791=CARTESIAN_POINT ( 'NONE',  ( -126.4213562373094959, -494.9999999999998863, 2.255140518769849223E-14 ) ) ;
#7815=ADVANCED_FACE ( 'NONE', ( #5264 ), #5328, .F. ) ;
#7830=DIRECTION ( 'NONE',  ( -0.000000000000000000, 1.000000000000000000, -0.000000000000000000 ) ) ;
#7843=LINE ( 'NONE', #5045, #7339 ) ;
#7847=CARTESIAN_POINT ( 'NONE',  ( 126.4213562373094959, -494.9999999999998863, 7.500000000000006217 ) ) ;
#7850=EDGE_CURVE ( 'NONE', #5193, #2379, #8554, .T. ) ;
#7855=CARTESIAN_POINT ( 'NONE',  ( 126.4213562373094959, -492.9999999999998863, -7.500000000000019540 ) ) ;
#7875=ORIENTED_EDGE ( 'NONE', *, *, #3978, .F. ) ;
#7885=ORIENTED_EDGE ( 'NONE', *, *, #1884, .F. ) ;
#7897=ORIENTED_EDGE ( 'NONE', *, *, #1790, .F. ) ;
#7918=CYLINDRICAL_SURFACE ( 'NONE', #9100, 7.500000000000012434 ) ;
#7928=DIRECTION ( 'NONE',  ( 0.000000000000000000, 0.000000000000000000, -1.000000000000000000 ) ) ;
#7933=ORIENTED_EDGE ( 'NONE', *, *, #8854, .T. ) ;
#7948=FACE_OUTER_BOUND ( 'NONE', #11646, .T. ) ;
#7955=DIRECTION ( 'NONE',  ( 1.000000000000000000, 0.000000000000000000, 0.000000000000000000 ) ) ;
#7971=EDGE_CURVE ( 'NONE', #11480, #5193, #4728, .T. ) ;
#7978=DIRECTION ( 'NONE',  ( 0.7071067811865477948, 0.000000000000000000, 0.7071067811865473507 ) ) ;
#7995=EDGE_CURVE ( 'NONE', #2379, #10867, #73, .T. ) ;
#8030=AXIS2_PLACEMENT_3D ( 'NONE', #8113, #11877, #3394 ) ;
#8040=CARTESIAN_POINT ( 'NONE',  ( 30.00000000000000000, -492.9999999999998863, -30.00000000000000000 ) ) ;
#8043=VECTOR ( 'NONE', #755, 1000.000000000000000 ) ;
#8064=CARTESIAN_POINT ( 'NONE',  ( 30.00000000000000000, -492.9999999999998863, 30.00000000000000000 ) ) ;
#8070=CIRCLE ( 'NONE', #8277, 7.500000000000007105 ) ;
#8075=DIRECTION ( 'NONE',  ( 0.000000000000000000, 0.000000000000000000, -1.000000000000000000 ) ) ;
#8082=AXIS2_PLACEMENT_3D ( 'NONE', #12056, #1742, #6248 ) ;
#8088=CIRCLE ( 'NONE', #2345, 7.500000000000007105 ) ;
#8108=EDGE_CURVE ( 'NONE', #2061, #5617, #5072, .T. ) ;
#8113=CARTESIAN_POINT ( 'NONE',  ( 126.4213562373094959, -494.9999999999998863, -6.938893903907228378E-15 ) ) ;
#8116=DIRECTION ( 'NONE',  ( -0.000000000000000000, 1.000000000000000000, -0.000000000000000000 ) ) ;
#8120=ORIENTED_EDGE ( 'NONE', *, *, #10896, .F. ) ;
#8129=LINE ( 'NONE', #6271, #11601 ) ;
#8130=AXIS2_PLACEMENT_3D ( 'NONE', #413, #1481, #9008 ) ;
#8131=VERTEX_POINT ( 'NONE', #6368 ) ;
#8146=DIRECTION ( 'NONE',  ( -0.000000000000000000, -0.000000000000000000, -1.000000000000000000 ) ) ;
#8147=MANIFOLD_SOLID_BREP ( 'Boss-Extrude8', #8295 ) ;
#8167=DIRECTION ( 'NONE',  ( 0.000000000000000000, 1.000000000000000000, 0.000000000000000000 ) ) ;
#8169=( NAMED_UNIT ( * ) PLANE_ANGLE_UNIT ( ) SI_UNIT ( $, .RADIAN. ) );
#8252=ORIENTED_EDGE ( 'NONE', *, *, #580, .T. ) ;
#8263=ORIENTED_EDGE ( 'NONE', *, *, #9793, .T. ) ;
#8268=ORIENTED_EDGE ( 'NONE', *, *, #7069, .F. ) ;
#8276=VECTOR ( 'NONE', #5840, 1000.000000000000000 ) ;
#8277=AXIS2_PLACEMENT_3D ( 'NONE', #3273, #9021, #7928 ) ;
#8283=DIRECTION ( 'NONE',  ( -0.7071067811865477948, 0.000000000000000000, -0.7071067811865473507 ) ) ;
#8295=CLOSED_SHELL ( 'NONE', ( #4952, #5307, #9692, #11010, #3393, #3437, #4866, #7143, #5156, #5488, #3754, #2138, #7350, #9192 ) ) ;
#8302=PLANE ( 'NONE',  #6004 ) ;
#8312=ORIENTED_EDGE ( 'NONE', *, *, #1495, .T. ) ;
#8313=ORIENTED_EDGE ( 'NONE', *, *, #4645, .T. ) ;
#8354=EDGE_LOOP ( 'NONE', ( #3032, #5825 ) ) ;
#8361=CIRCLE ( 'NONE', #1241, 7.500000000000007105 ) ;
#8367=DIRECTION ( 'NONE',  ( 0.000000000000000000, 0.000000000000000000, -1.000000000000000000 ) ) ;
#8392=DIRECTION ( 'NONE',  ( -0.7071067811865473507, 0.000000000000000000, 0.7071067811865477948 ) ) ;
#8406=CARTESIAN_POINT ( 'NONE',  ( -30.00000000000000000, -492.9999999999998863, 30.00000000000000000 ) ) ;
#8429=EDGE_LOOP ( 'NONE', ( #4124, #11504, #12165, #11569 ) ) ;
#8483=CARTESIAN_POINT ( 'NONE',  ( -30.00000000000000000, -492.9999999999998863, -30.00000000000000000 ) ) ;
#8488=DIRECTION ( 'NONE',  ( -0.000000000000000000, 1.000000000000000000, -0.000000000000000000 ) ) ;
#8505=LINE ( 'NONE', #5525, #1450 ) ;
#8543=CYLINDRICAL_SURFACE ( 'NONE', #7349, 7.500000000000007105 ) ;
#8554=LINE ( 'NONE', #10281, #2141 ) ;
#8580=CYLINDRICAL_SURFACE ( 'NONE', #661, 7.500000000000012434 ) ;
#8619=PRODUCT ( 'Cast Iron Base Mounting Frame', 'Cast Iron Base Mounting Frame', '', ( #1094 ) ) ;
#8625=AXIS2_PLACEMENT_3D ( 'NONE', #10040, #11777, #9858 ) ;
#8630=VERTEX_POINT ( 'NONE', #5787 ) ;
#8723=EDGE_LOOP ( 'NONE', ( #6572, #3893, #11873, #7875 ) ) ;
#8748=EDGE_LOOP ( 'NONE', ( #4503, #10534, #9765, #5974 ) ) ;
#8771=FACE_BOUND ( 'NONE', #1831, .T. ) ;
#8799=FACE_OUTER_BOUND ( 'NONE', #6891, .T. ) ;
#8803=VERTEX_POINT ( 'NONE', #5770 ) ;
#8812=UNCERTAINTY_MEASURE_WITH_UNIT (LENGTH_MEASURE( 1.000000000000000082E-05 ), #2722, 'distance_accuracy_value', 'NONE');
#8834=DIRECTION ( 'NONE',  ( 0.000000000000000000, 0.000000000000000000, 1.000000000000000000 ) ) ;
#8848=DIRECTION ( 'NONE',  ( -0.000000000000000000, 1.000000000000000000, -0.000000000000000000 ) ) ;
#8854=EDGE_CURVE ( 'NONE', #5617, #8131, #8070, .T. ) ;
#8889=PLANE ( 'NONE',  #9908 ) ;
#8908=EDGE_CURVE ( 'NONE', #4868, #6384, #9282, .T. ) ;
#8912=DIRECTION ( 'NONE',  ( 0.000000000000000000, 0.000000000000000000, -1.000000000000000000 ) ) ;
#8935=CARTESIAN_POINT ( 'NONE',  ( 28.00000000000000000, -492.9999999999998863, -27.99999999999999645 ) ) ;
#8950=EDGE_LOOP ( 'NONE', ( #12220, #4739, #5143, #5139 ) ) ;
#8972=DIRECTION ( 'NONE',  ( -0.000000000000000000, 0.000000000000000000, 1.000000000000000000 ) ) ;
#8985=SHAPE_REPRESENTATION_RELATIONSHIP ( 'NONE' , 'NONE' ,  #3601, #3830 ) ;
#8996=ADVANCED_FACE ( 'NONE', ( #10324, #2662 ), #7306, .T. ) ;
#9008=DIRECTION ( 'NONE',  ( 0.000000000000000000, 0.000000000000000000, -1.000000000000000000 ) ) ;
#9021=DIRECTION ( 'NONE',  ( 0.000000000000000000, -1.000000000000000000, 0.000000000000000000 ) ) ;
#9039=LINE ( 'NONE', #706, #256 ) ;
#9048=CARTESIAN_POINT ( 'NONE',  ( 0.000000000000000000, 0.000000000000000000, 0.000000000000000000 ) ) ;
#9050=DIRECTION ( 'NONE',  ( 0.000000000000000000, -0.000000000000000000, 1.000000000000000000 ) ) ;
#9052=DIRECTION ( 'NONE',  ( -0.000000000000000000, 1.000000000000000000, -0.000000000000000000 ) ) ;
#9067=VERTEX_POINT ( 'NONE', #9147 ) ;
#9080=FILL_AREA_STYLE ('',( #7360 ) ) ;
#9083=FILL_AREA_STYLE_COLOUR ( '', #10224 ) ;
#9085=EDGE_CURVE ( 'NONE', #7650, #5299, #7274, .T. ) ;
#9096=ORIENTED_EDGE ( 'NONE', *, *, #7386, .F. ) ;
#9100=AXIS2_PLACEMENT_3D ( 'NONE', #7791, #1361, #8834 ) ;
#9106=CARTESIAN_POINT ( 'NONE',  ( -27.99999999999999645, -492.9999999999998863, 27.99999999999999645 ) ) ;
#9143=DIRECTION ( 'NONE',  ( -0.000000000000000000, 0.000000000000000000, -1.000000000000000000 ) ) ;
#9147=CARTESIAN_POINT ( 'NONE',  ( 27.99999999999999645, -6.000000000000000000, 28.00000000000000000 ) ) ;
#9152=EDGE_LOOP ( 'NONE', ( #4365, #6204, #9177, #3445 ) ) ;
#9163=CARTESIAN_POINT ( 'NONE',  ( 1.479627290717497352E-14, -494.9999999999998863, 118.9213562373094817 ) ) ;
#9168=CIRCLE ( 'NONE', #2658, 7.500000000000012434 ) ;
#9177=ORIENTED_EDGE ( 'NONE', *, *, #8908, .T. ) ;
#9192=ADVANCED_FACE ( 'NONE', ( #1473 ), #9819, .F. ) ;
#9212=LINE ( 'NONE', #12059, #3060 ) ;
#9215=VERTEX_POINT ( 'NONE', #3317 ) ;
#9216=LINE ( 'NONE', #7533, #8043 ) ;
#9227=DIRECTION ( 'NONE',  ( -0.000000000000000000, -0.000000000000000000, -1.000000000000000000 ) ) ;
#9269=ORIENTED_EDGE ( 'NONE', *, *, #5555, .T. ) ;
#9282=LINE ( 'NONE', #10207, #2745 ) ;
#9298=CARTESIAN_POINT ( 'NONE',  ( 27.99999999999999645, -492.9999999999998863, 27.99999999999999645 ) ) ;
#9322=CARTESIAN_POINT ( 'NONE',  ( 126.4213562373094959, -494.9999999999998863, -7.500000000000019540 ) ) ;
#9328=VECTOR ( 'NONE', #7166, 1000.000000000000000 ) ;
#9337=PRESENTATION_STYLE_ASSIGNMENT (( #5562 ) ) ;
#9338=CARTESIAN_POINT ( 'NONE',  ( -27.99999999999999645, -492.9999999999998863, -27.99999999999999645 ) ) ;
#9340=EDGE_CURVE ( 'NONE', #11012, #4868, #4442, .T. ) ;
#9372=AXIS2_PLACEMENT_3D ( 'NONE', #3619, #665, #8283 ) ;
#9373=VECTOR ( 'NONE', #11836, 1000.000000000000000 ) ;
#9378=CARTESIAN_POINT ( 'NONE',  ( -27.99999999999999645, -492.9999999999998863, 27.99999999999999645 ) ) ;
#9408=EDGE_CURVE ( 'NONE', #1622, #7207, #3466, .T. ) ;
#9421=EDGE_CURVE ( 'NONE', #7650, #1611, #9974, .T. ) ;
#9428=FACE_OUTER_BOUND ( 'NONE', #2796, .T. ) ;
#9434=ORIENTED_EDGE ( 'NONE', *, *, #3959, .T. ) ;
#9456=FACE_OUTER_BOUND ( 'NONE', #4970, .T. ) ;
#9490=CARTESIAN_POINT ( 'NONE',  ( -141.4213562373095101, -492.9999999999998863, 3.644282033693712520E-14 ) ) ;
#9503=FACE_OUTER_BOUND ( 'NONE', #8429, .T. ) ;
#9578=PLANE ( 'NONE',  #2153 ) ;
#9587=CARTESIAN_POINT ( 'NONE',  ( 1.387778780781445676E-14, -494.9999999999998863, 133.9213562373095101 ) ) ;
#9599=ORIENTED_EDGE ( 'NONE', *, *, #1026, .T. ) ;
#9641=CARTESIAN_POINT ( 'NONE',  ( 1.479627290717497352E-14, -492.9999999999998863, 118.9213562373094817 ) ) ;
#9645=EDGE_CURVE ( 'NONE', #5463, #11262, #5077, .T. ) ;
#9658=DIRECTION ( 'NONE',  ( 0.000000000000000000, 0.000000000000000000, -1.000000000000000000 ) ) ;
#9683=ORIENTED_EDGE ( 'NONE', *, *, #5555, .F. ) ;
#9690=ORIENTED_EDGE ( 'NONE', *, *, #4645, .F. ) ;
#9692=ADVANCED_FACE ( 'NONE', ( #565 ), #4345, .F. ) ;
#9697=LINE ( 'NONE', #1238, #5822 ) ;
#9699=FACE_OUTER_BOUND ( 'NONE', #7752, .T. ) ;
#9708=ORIENTED_EDGE ( 'NONE', *, *, #11442, .F. ) ;
#9715=ADVANCED_FACE ( 'NONE', ( #7948 ), #510, .F. ) ;
#9734=CARTESIAN_POINT ( 'NONE',  ( 0.000000000000000000, -494.9999999999998863, -118.9213562373094817 ) ) ;
#9765=ORIENTED_EDGE ( 'NONE', *, *, #11081, .T. ) ;
#9767=AXIS2_PLACEMENT_3D ( 'NONE', #2562, #9052, #3200 ) ;
#9782=DIRECTION ( 'NONE',  ( -0.000000000000000000, 0.000000000000000000, -1.000000000000000000 ) ) ;
#9793=EDGE_CURVE ( 'NONE', #4581, #3571, #4233, .T. ) ;
#9795=UNCERTAINTY_MEASURE_WITH_UNIT (LENGTH_MEASURE( 1.000000000000000082E-05 ), #4176, 'distance_accuracy_value', 'NONE');
#9819=CYLINDRICAL_SURFACE ( 'NONE', #1144, 7.500000000000012434 ) ;
#9857=CLOSED_SHELL ( 'NONE', ( #6987, #8996, #9715, #7815, #1048, #3289, #6596, #10881, #10071, #6667 ) ) ;
#9858=DIRECTION ( 'NONE',  ( 0.000000000000000000, 0.000000000000000000, 1.000000000000000000 ) ) ;
#9890=ORIENTED_EDGE ( 'NONE', *, *, #8108, .T. ) ;
#9899=VECTOR ( 'NONE', #8392, 999.9999999999998863 ) ;
#9908=AXIS2_PLACEMENT_3D ( 'NONE', #10812, #2402, #7978 ) ;
#9911=DIRECTION ( 'NONE',  ( 0.000000000000000000, 0.000000000000000000, -1.000000000000000000 ) ) ;
#9965=CARTESIAN_POINT ( 'NONE',  ( -6.360897667028196044E-14, -494.9999999999998863, -141.4213562373094817 ) ) ;
#9974=LINE ( 'NONE', #9163, #3086 ) ;
#9982=ORIENTED_EDGE ( 'NONE', *, *, #10704, .T. ) ;
#9985=FACE_OUTER_BOUND ( 'NONE', #9152, .T. ) ;
#9988=CARTESIAN_POINT ( 'NONE',  ( -6.360897667028196044E-14, -492.9999999999998863, -141.4213562373094817 ) ) ;
#10029=ORIENTED_EDGE ( 'NONE', *, *, #11739, .T. ) ;
#10040=CARTESIAN_POINT ( 'NONE',  ( 30.00000000000000000, -492.9999999999998863, -30.00000000000000000 ) ) ;
#10071=ADVANCED_FACE ( 'NONE', ( #436 ), #6009, .T. ) ;
#10073=FACE_OUTER_BOUND ( 'NONE', #2919, .T. ) ;
#10088=EDGE_LOOP ( 'NONE', ( #5062, #7933 ) ) ;
#10120=ORIENTED_EDGE ( 'NONE', *, *, #4672, .T. ) ;
#10168=VERTEX_POINT ( 'NONE', #7242 ) ;
#10182=EDGE_LOOP ( 'NONE', ( #8313, #11465, #7786, #9708 ) ) ;
#10206=CARTESIAN_POINT ( 'NONE',  ( -141.4213562373095101, -492.9999999999998863, 3.644282033693712520E-14 ) ) ;
#10207=CARTESIAN_POINT ( 'NONE',  ( -30.00000000000000000, -492.9999999999998863, -30.00000000000000000 ) ) ;
#10217=ORIENTED_EDGE ( 'NONE', *, *, #11888, .F. ) ;
#10224=COLOUR_RGB ( '', 0.66274510, 0.83137255, 0.94901961) ;
#10231=DIRECTION ( 'NONE',  ( 0.000000000000000000, 0.000000000000000000, 1.000000000000000000 ) ) ;
#10244=AXIS2_PLACEMENT_3D ( 'NONE', #10678, #10620, #5739 ) ;
#10249=EDGE_CURVE ( 'NONE', #1735, #8803, #9216, .T. ) ;
#10271=CARTESIAN_POINT ( 'NONE',  ( 0.000000000000000000, -6.000000000000000000, 0.000000000000000000 ) ) ;
#10281=CARTESIAN_POINT ( 'NONE',  ( -141.4213562373095101, -494.9999999999998863, 3.644282033693712520E-14 ) ) ;
#10324=FACE_OUTER_BOUND ( 'NONE', #12069, .T. ) ;
#10332=VERTEX_POINT ( 'NONE', #507 ) ;
#10342=ORIENTED_EDGE ( 'NONE', *, *, #12116, .T. ) ;
#10375=EDGE_CURVE ( 'NONE', #1167, #6680, #10911, .T. ) ;
#10423=DIRECTION ( 'NONE',  ( 0.000000000000000000, -1.000000000000000000, 0.000000000000000000 ) ) ;
#10447=ORIENTED_EDGE ( 'NONE', *, *, #7995, .T. ) ;
#10507=DIRECTION ( 'NONE',  ( -0.000000000000000000, 1.000000000000000000, -0.000000000000000000 ) ) ;
#10534=ORIENTED_EDGE ( 'NONE', *, *, #11249, .T. ) ;
#10535=SHAPE_DEFINITION_REPRESENTATION ( #11481, #3601 ) ;
#10567=DIRECTION ( 'NONE',  ( 6.195440985631454085E-17, 0.000000000000000000, -1.000000000000000000 ) ) ;
#10594=AXIS2_PLACEMENT_3D ( 'NONE', #2300, #11423, #40 ) ;
#10620=DIRECTION ( 'NONE',  ( 0.000000000000000000, -1.000000000000000000, 0.000000000000000000 ) ) ;
#10654=CARTESIAN_POINT ( 'NONE',  ( 28.00000000000000000, -6.000000000000000000, -27.99999999999999645 ) ) ;
#10662=LINE ( 'NONE', #9734, #1095 ) ;
#10678=CARTESIAN_POINT ( 'NONE',  ( 0.000000000000000000, -492.9999999999998863, 0.000000000000000000 ) ) ;
#10683=VERTEX_POINT ( 'NONE', #4359 ) ;
#10700=CARTESIAN_POINT ( 'NONE',  ( -126.4213562373094959, -492.9999999999998863, -7.499999999999990230 ) ) ;
#10704=EDGE_CURVE ( 'NONE', #11382, #7316, #8129, .T. ) ;
#10708=ORIENTED_EDGE ( 'NONE', *, *, #5752, .F. ) ;
#10712=PLANE ( 'NONE',  #10944 ) ;
#10714=DIRECTION ( 'NONE',  ( 0.000000000000000000, -1.000000000000000000, 0.000000000000000000 ) ) ;
#10771=DIRECTION ( 'NONE',  ( 1.000000000000000000, 0.000000000000000000, 0.000000000000000000 ) ) ;
#10779=EDGE_CURVE ( 'NONE', #11480, #11382, #4539, .T. ) ;
#10812=CARTESIAN_POINT ( 'NONE',  ( -6.360897667028196044E-14, -494.9999999999998863, -141.4213562373094817 ) ) ;
#10814=VECTOR ( 'NONE', #594, 1000.000000000000000 ) ;
#10819=CARTESIAN_POINT ( 'NONE',  ( -126.4213562373094959, -494.9999999999998863, -7.499999999999990230 ) ) ;
#10833=DIRECTION ( 'NONE',  ( 0.000000000000000000, -1.000000000000000000, 0.000000000000000000 ) ) ;
#10866=ORIENTED_EDGE ( 'NONE', *, *, #10896, .T. ) ;
#10867=VERTEX_POINT ( 'NONE', #4221 ) ;
#10877=SURFACE_STYLE_FILL_AREA ( #623 ) ;
#10881=ADVANCED_FACE ( 'NONE', ( #6942 ), #10712, .T. ) ;
#10887=DIRECTION ( 'NONE',  ( -0.000000000000000000, 1.000000000000000000, -0.000000000000000000 ) ) ;
#10896=EDGE_CURVE ( 'NONE', #3571, #10683, #6017, .T. ) ;
#10904=DIRECTION ( 'NONE',  ( 0.000000000000000000, 0.000000000000000000, 1.000000000000000000 ) ) ;
#10907=EDGE_CURVE ( 'NONE', #5463, #11012, #778, .T. ) ;
#10911=LINE ( 'NONE', #9988, #2122 ) ;
#10929=DIRECTION ( 'NONE',  ( 0.7071067811865473507, 0.000000000000000000, -0.7071067811865477948 ) ) ;
#10942=CIRCLE ( 'NONE', #4239, 7.500000000000012434 ) ;
#10943=CARTESIAN_POINT ( 'NONE',  ( -30.00000000000000000, -492.9999999999998863, -30.00000000000000000 ) ) ;
#10944=AXIS2_PLACEMENT_3D ( 'NONE', #11827, #8972, #10771 ) ;
#10988=DIRECTION ( 'NONE',  ( -1.000000000000000000, -0.000000000000000000, -0.000000000000000000 ) ) ;
#11006=VECTOR ( 'NONE', #1941, 999.9999999999998863 ) ;
#11010=ADVANCED_FACE ( 'NONE', ( #9428 ), #17, .F. ) ;
#11012=VERTEX_POINT ( 'NONE', #1207 ) ;
#11015=ORIENTED_EDGE ( 'NONE', *, *, #10779, .F. ) ;
#11050=ORIENTED_EDGE ( 'NONE', *, *, #4512, .T. ) ;
#11055=CARTESIAN_POINT ( 'NONE',  ( 0.000000000000000000, -494.9999999999998863, -118.9213562373094817 ) ) ;
#11081=EDGE_CURVE ( 'NONE', #11517, #8131, #10662, .T. ) ;
#11145=VECTOR ( 'NONE', #781, 1000.000000000000000 ) ;
#11176=VECTOR ( 'NONE', #11344, 999.9999999999998863 ) ;
#11189=CARTESIAN_POINT ( 'NONE',  ( 141.4213562373095101, -494.9999999999998863, -1.508194112741312283E-14 ) ) ;
#11220=CARTESIAN_POINT ( 'NONE',  ( 4.808665244885994618E-14, -494.9999999999998863, 141.4213562373094817 ) ) ;
#11233=EDGE_CURVE ( 'NONE', #8803, #6402, #9168, .T. ) ;
#11241=PLANE ( 'NONE',  #1034 ) ;
#11249=EDGE_CURVE ( 'NONE', #2061, #11517, #7790, .T. ) ;
#11262=VERTEX_POINT ( 'NONE', #3470 ) ;
#11263=DIRECTION ( 'NONE',  ( -0.000000000000000000, -0.000000000000000000, -1.000000000000000000 ) ) ;
#11265=ORIENTED_EDGE ( 'NONE', *, *, #7971, .F. ) ;
#11277=EDGE_CURVE ( 'NONE', #11012, #9215, #7130, .T. ) ;
#11289=DIRECTION ( 'NONE',  ( -1.000000000000000000, -0.000000000000000000, -6.195440985631455317E-17 ) ) ;
#11295=CARTESIAN_POINT ( 'NONE',  ( 126.4213562373094959, -494.9999999999998863, -6.938893903907228378E-15 ) ) ;
#11313=CARTESIAN_POINT ( 'NONE',  ( -27.99999999999999645, -492.9999999999998863, 27.99999999999999645 ) ) ;
#11319=DIRECTION ( 'NONE',  ( 1.000000000000000000, 0.000000000000000000, 0.000000000000000000 ) ) ;
#11344=DIRECTION ( 'NONE',  ( 0.7071067811865473507, 0.000000000000000000, -0.7071067811865477948 ) ) ;
#11345=CARTESIAN_POINT ( 'NONE',  ( 126.4213562373094959, -492.9999999999998863, -6.938893903907228378E-15 ) ) ;
#11351=PRODUCT_DEFINITION_CONTEXT ( 'detailed design', #11822, 'design' ) ;
#11366=ORIENTED_EDGE ( 'NONE', *, *, #6220, .F. ) ;
#11370=FACE_BOUND ( 'NONE', #10088, .T. ) ;
#11372=LINE ( 'NONE', #1921, #1463 ) ;
#11382=VERTEX_POINT ( 'NONE', #577 ) ;
#11423=DIRECTION ( 'NONE',  ( -1.000000000000000000, 0.000000000000000000, -6.195440985631454085E-17 ) ) ;
#11428=ORIENTED_EDGE ( 'NONE', *, *, #9645, .F. ) ;
#11442=EDGE_CURVE ( 'NONE', #1342, #7207, #7323, .T. ) ;
#11455=EDGE_LOOP ( 'NONE', ( #9269, #12161, #6441, #3879 ) ) ;
#11465=ORIENTED_EDGE ( 'NONE', *, *, #6843, .T. ) ;
#11468=CARTESIAN_POINT ( 'NONE',  ( 126.4213562373094959, -492.9999999999998863, 7.500000000000006217 ) ) ;
#11480=VERTEX_POINT ( 'NONE', #541 ) ;
#11481=PRODUCT_DEFINITION_SHAPE ( 'NONE', 'NONE',  #3143 ) ;
#11495=DIRECTION ( 'NONE',  ( 0.000000000000000000, 0.000000000000000000, -1.000000000000000000 ) ) ;
#11504=ORIENTED_EDGE ( 'NONE', *, *, #6937, .T. ) ;
#11517=VERTEX_POINT ( 'NONE', #11055 ) ;
#11545=AXIS2_PLACEMENT_3D ( 'NONE', #1514, #5276, #9050 ) ;
#11548=ORIENTED_EDGE ( 'NONE', *, *, #3959, .F. ) ;
#11552=VECTOR ( 'NONE', #5895, 1000.000000000000000 ) ;
#11561=CARTESIAN_POINT ( 'NONE',  ( 126.4213562373094959, -494.9999999999998863, -6.938893903907228378E-15 ) ) ;
#11569=ORIENTED_EDGE ( 'NONE', *, *, #9408, .F. ) ;
#11592=APPLICATION_CONTEXT ( 'automotive_design' ) ;
#11601=VECTOR ( 'NONE', #11892, 999.9999999999998863 ) ;
#11646=EDGE_LOOP ( 'NONE', ( #6139, #1747, #3700, #358 ) ) ;
#11658=CARTESIAN_POINT ( 'NONE',  ( 126.4213562373094959, -494.9999999999998863, -6.938893903907228378E-15 ) ) ;
#11660=UNCERTAINTY_MEASURE_WITH_UNIT (LENGTH_MEASURE( 1.000000000000000082E-05 ), #752, 'distance_accuracy_value', 'NONE');
#11739=EDGE_CURVE ( 'NONE', #7713, #9067, #9212, .T. ) ;
#11760=CARTESIAN_POINT ( 'NONE',  ( -27.99999999999999645, -6.000000000000000000, -27.99999999999999645 ) ) ;
#11777=DIRECTION ( 'NONE',  ( -1.000000000000000000, 0.000000000000000000, 0.000000000000000000 ) ) ;
#11791=DIRECTION ( 'NONE',  ( -1.000000000000000000, -0.000000000000000000, -6.195440985631455317E-17 ) ) ;
#11822=APPLICATION_CONTEXT ( 'automotive_design' ) ;
#11827=CARTESIAN_POINT ( 'NONE',  ( -27.99999999999999645, -492.9999999999998863, -27.99999999999999645 ) ) ;
#11830=MECHANICAL_DESIGN_GEOMETRIC_PRESENTATION_REPRESENTATION('',(#3324),#2162);
#11836=DIRECTION ( 'NONE',  ( -0.000000000000000000, 1.000000000000000000, -0.000000000000000000 ) ) ;
#11873=ORIENTED_EDGE ( 'NONE', *, *, #10249, .T. ) ;
#11877=DIRECTION ( 'NONE',  ( -0.000000000000000000, 1.000000000000000000, -0.000000000000000000 ) ) ;
#11888=EDGE_CURVE ( 'NONE', #9215, #10168, #9697, .T. ) ;
#11892=DIRECTION ( 'NONE',  ( -0.7071067811865479058, 0.000000000000000000, -0.7071067811865472397 ) ) ;
#11896=PLANE ( 'NONE',  #11545 ) ;
#11916=CARTESIAN_POINT ( 'NONE',  ( -30.00000000000000000, -492.9999999999998863, 30.00000000000000000 ) ) ;
#11918=DIRECTION ( 'NONE',  ( -0.7071067811865473507, 0.000000000000000000, 0.7071067811865477948 ) ) ;
#11935=ORIENTED_EDGE ( 'NONE', *, *, #5319, .T. ) ;
#11957=AXIS2_PLACEMENT_3D ( 'NONE', #9048, #10904, #7955 ) ;
#11963=ORIENTED_EDGE ( 'NONE', *, *, #7191, .T. ) ;
#11965=LINE ( 'NONE', #2627, #10814 ) ;
#11982=CARTESIAN_POINT ( 'NONE',  ( -141.4213562373095101, -494.9999999999998863, 3.644282033693712520E-14 ) ) ;
#11990=DIRECTION ( 'NONE',  ( 1.000000000000000000, 0.000000000000000000, -0.000000000000000000 ) ) ;
#12025=CYLINDRICAL_SURFACE ( 'NONE', #9767, 7.500000000000007105 ) ;
#12032=CARTESIAN_POINT ( 'NONE',  ( -126.4213562373094959, -494.9999999999998863, 7.500000000000035527 ) ) ;
#12056=CARTESIAN_POINT ( 'NONE',  ( 0.000000000000000000, -494.9999999999998863, -126.4213562373094959 ) ) ;
#12059=CARTESIAN_POINT ( 'NONE',  ( 27.99999999999999645, -492.9999999999998863, 28.00000000000000000 ) ) ;
#12069=EDGE_LOOP ( 'NONE', ( #3389, #3279, #9096, #10217 ) ) ;
#12073=CARTESIAN_POINT ( 'NONE',  ( -30.00000000000000000, -6.000000000000000000, -30.00000000000000000 ) ) ;
#12076=ORIENTED_EDGE ( 'NONE', *, *, #2267, .F. ) ;
#12101=CARTESIAN_POINT ( 'NONE',  ( 9.184850993605165694E-16, -492.9999999999998863, -133.9213562373095101 ) ) ;
#12116=EDGE_CURVE ( 'NONE', #7316, #1167, #2885, .T. ) ;
#12126=( NAMED_UNIT ( * ) PLANE_ANGLE_UNIT ( ) SI_UNIT ( $, .RADIAN. ) );
#12161=ORIENTED_EDGE ( 'NONE', *, *, #9421, .T. ) ;
#12165=ORIENTED_EDGE ( 'NONE', *, *, #11442, .T. ) ;
#12170=FACE_OUTER_BOUND ( 'NONE', #5608, .T. ) ;
#12184=ORIENTED_EDGE ( 'NONE', *, *, #7191, .F. ) ;
#12192=DIRECTION ( 'NONE',  ( 1.000000000000000000, 0.000000000000000000, -0.000000000000000000 ) ) ;
#12220=ORIENTED_EDGE ( 'NONE', *, *, #11888, .T. ) ;
#12225=AXIS2_PLACEMENT_3D ( 'NONE', #8483, #1917, #112 ) ;
ENDSEC;
END-ISO-10303-21;
